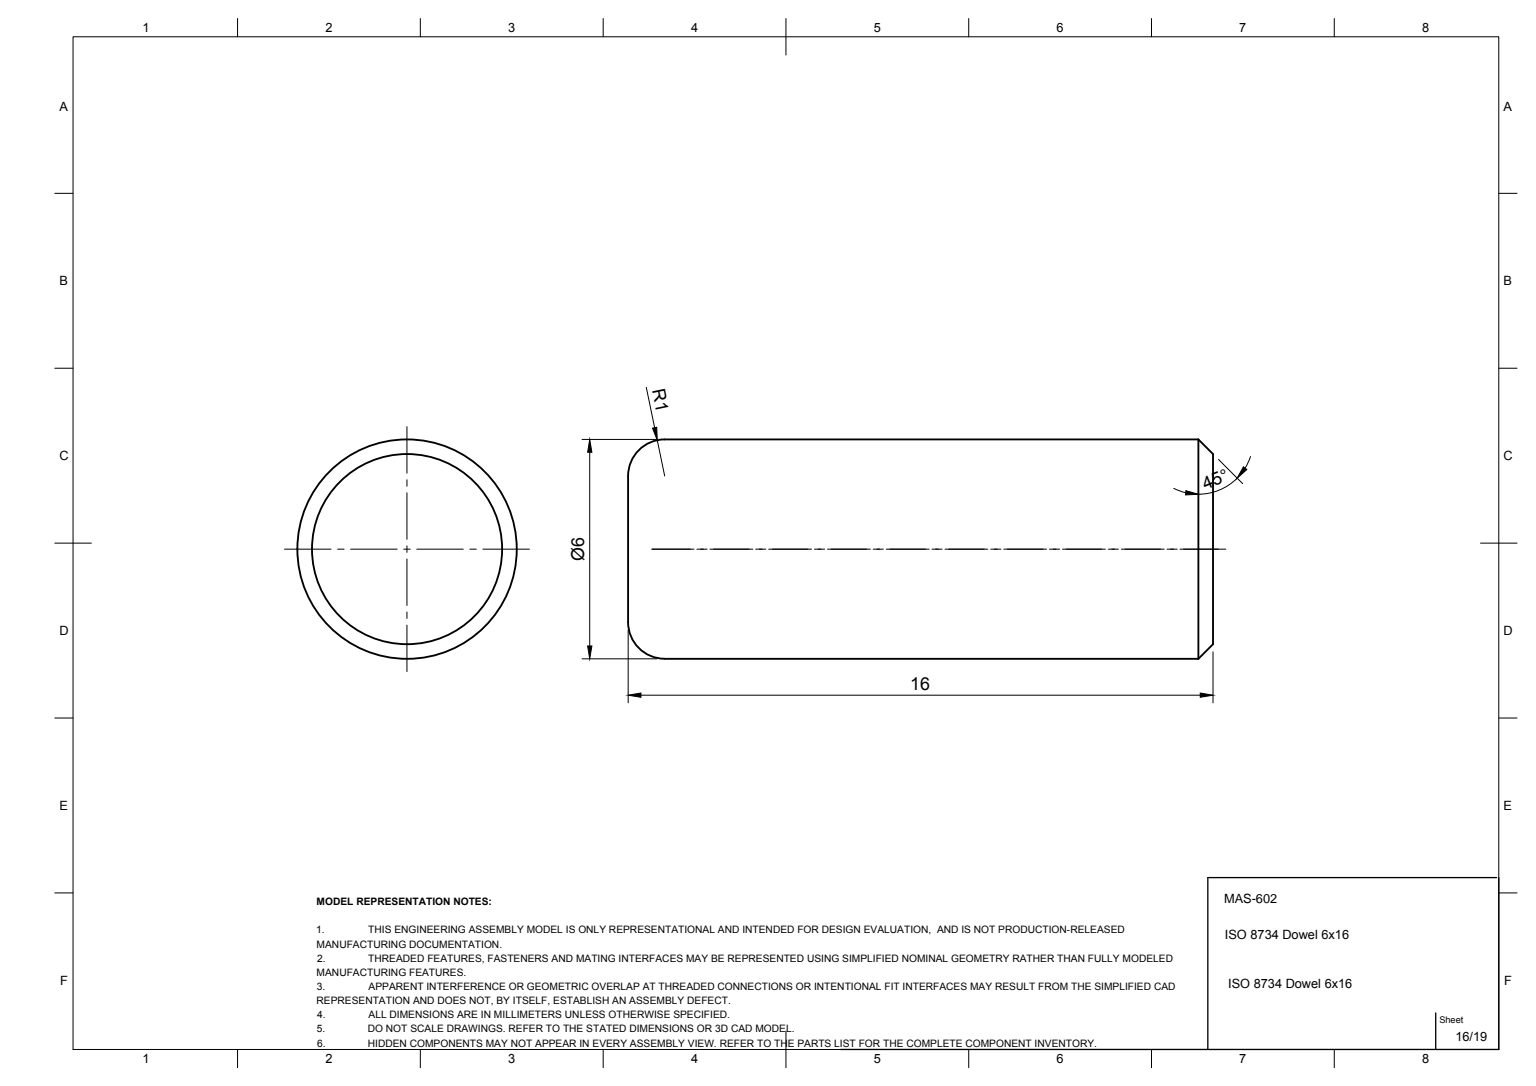
ISO-10303-21;
HEADER;
/* Generated by software containing ST-Developer
 * from STEP Tools, Inc. (www.steptools.com) 
 */

FILE_DESCRIPTION(
/* description */ (''),
/* implementation_level */ '2;1');

FILE_NAME(
/* name */ 'ISO 8734 Dowel 6x16.step',
/* time_stamp */ '2026-10-15T14:42:47-07:00',
/* author */ (''),
/* organization */ (''),
/* preprocessor_version */ 'ST-DEVELOPER v20.2',
/* originating_system */ 'Autodesk Translation Framework v15.15.0.0',
/* authorisation */ '');

FILE_SCHEMA (('AUTOMOTIVE_DESIGN { 1 0 10303 214 3 1 1 }'));
ENDSEC;

DATA;
#10=MECHANICAL_DESIGN_GEOMETRIC_PRESENTATION_REPRESENTATION('',(#248),#85789);
#189=CONICAL_SURFACE('',#10787,0.28,0.785398163397448);
#212=SHAPE_REPRESENTATION_RELATIONSHIP('SRR','None',#85877,#230);
#230=ADVANCED_BREP_SHAPE_REPRESENTATION('',(#266),#85785);
#248=STYLED_ITEM('',(#85976),#266);
#266=MANIFOLD_SOLID_BREP('Body1',#9895);
#1175=PLANE('',#10784);
#1176=PLANE('',#10785);
#1660=LINE('',#77882,#2196);
#1661=LINE('',#77889,#2197);
#2196=VECTOR('',#12790,0.3);
#2197=VECTOR('',#12801,0.28);
#2364=CYLINDRICAL_SURFACE('',#10782,0.3);
#2828=FACE_OUTER_BOUND('',#3416,.T.);
#2829=FACE_OUTER_BOUND('',#3417,.T.);
#2830=FACE_OUTER_BOUND('',#3418,.T.);
#2831=FACE_OUTER_BOUND('',#3419,.T.);
#2832=FACE_OUTER_BOUND('',#3420,.T.);
#3416=EDGE_LOOP('',(#8889,#8890,#8891,#8892));
#3417=EDGE_LOOP('',(#8893,#8894,#8895,#8896));
#3418=EDGE_LOOP('',(#8897));
#3419=EDGE_LOOP('',(#8898));
#3420=EDGE_LOOP('',(#8899,#8900,#8901,#8902));
#3820=CIRCLE('',#10779,0.2);
#3821=CIRCLE('',#10780,0.1);
#3822=CIRCLE('',#10781,0.3);
#3823=CIRCLE('',#10783,0.3);
#3824=CIRCLE('',#10786,0.26);
#4757=VERTEX_POINT('',#77875);
#4758=VERTEX_POINT('',#77877);
#4759=VERTEX_POINT('',#77881);
#4760=VERTEX_POINT('',#77886);
#6172=EDGE_CURVE('',#4757,#4757,#3820,.T.);
#6173=EDGE_CURVE('',#4757,#4758,#3821,.T.);
#6174=EDGE_CURVE('',#4758,#4758,#3822,.T.);
#6175=EDGE_CURVE('',#4758,#4759,#1660,.T.);
#6176=EDGE_CURVE('',#4759,#4759,#3823,.T.);
#6177=EDGE_CURVE('',#4760,#4760,#3824,.T.);
#6178=EDGE_CURVE('',#4759,#4760,#1661,.T.);
#8889=ORIENTED_EDGE('',*,*,#6172,.T.);
#8890=ORIENTED_EDGE('',*,*,#6173,.T.);
#8891=ORIENTED_EDGE('',*,*,#6174,.T.);
#8892=ORIENTED_EDGE('',*,*,#6173,.F.);
#8893=ORIENTED_EDGE('',*,*,#6174,.F.);
#8894=ORIENTED_EDGE('',*,*,#6175,.T.);
#8895=ORIENTED_EDGE('',*,*,#6176,.T.);
#8896=ORIENTED_EDGE('',*,*,#6175,.F.);
#8897=ORIENTED_EDGE('',*,*,#6172,.F.);
#8898=ORIENTED_EDGE('',*,*,#6177,.F.);
#8899=ORIENTED_EDGE('',*,*,#6176,.F.);
#8900=ORIENTED_EDGE('',*,*,#6178,.T.);
#8901=ORIENTED_EDGE('',*,*,#6177,.T.);
#8902=ORIENTED_EDGE('',*,*,#6178,.F.);
#9379=TOROIDAL_SURFACE('',#10778,0.2,0.1);
#9806=ADVANCED_FACE('',(#2828),#9379,.T.);
#9807=ADVANCED_FACE('',(#2829),#2364,.T.);
#9808=ADVANCED_FACE('',(#2830),#1175,.T.);
#9809=ADVANCED_FACE('',(#2831),#1176,.T.);
#9810=ADVANCED_FACE('',(#2832),#189,.T.);
#9895=CLOSED_SHELL('',(#9806,#9807,#9808,#9809,#9810));
#10777=AXIS2_PLACEMENT_3D('',#77873,#12778,#12779);
#10778=AXIS2_PLACEMENT_3D('',#77874,#12780,#12781);
#10779=AXIS2_PLACEMENT_3D('',#77876,#12782,#12783);
#10780=AXIS2_PLACEMENT_3D('',#77878,#12784,#12785);
#10781=AXIS2_PLACEMENT_3D('',#77879,#12786,#12787);
#10782=AXIS2_PLACEMENT_3D('',#77880,#12788,#12789);
#10783=AXIS2_PLACEMENT_3D('',#77883,#12791,#12792);
#10784=AXIS2_PLACEMENT_3D('',#77884,#12793,#12794);
#10785=AXIS2_PLACEMENT_3D('',#77885,#12795,#12796);
#10786=AXIS2_PLACEMENT_3D('',#77887,#12797,#12798);
#10787=AXIS2_PLACEMENT_3D('',#77888,#12799,#12800);
#12778=DIRECTION('axis',(0.,0.,1.));
#12779=DIRECTION('refdir',(1.,0.,0.));
#12780=DIRECTION('center_axis',(0.,0.,1.));
#12781=DIRECTION('ref_axis',(1.,0.,0.));
#12782=DIRECTION('center_axis',(0.,0.,-1.));
#12783=DIRECTION('ref_axis',(-1.,1.22464679914735E-16,0.));
#12784=DIRECTION('center_axis',(1.22464679914735E-16,-1.,0.));
#12785=DIRECTION('ref_axis',(-1.,-1.22464679914735E-16,0.));
#12786=DIRECTION('center_axis',(0.,0.,1.));
#12787=DIRECTION('ref_axis',(-1.,1.22464679914735E-16,0.));
#12788=DIRECTION('center_axis',(0.,0.,1.));
#12789=DIRECTION('ref_axis',(1.,0.,0.));
#12790=DIRECTION('',(0.,0.,-1.));
#12791=DIRECTION('center_axis',(0.,0.,1.));
#12792=DIRECTION('ref_axis',(1.,0.,0.));
#12793=DIRECTION('center_axis',(0.,0.,1.));
#12794=DIRECTION('ref_axis',(1.,0.,0.));
#12795=DIRECTION('center_axis',(0.,0.,-1.));
#12796=DIRECTION('ref_axis',(-1.,0.,0.));
#12797=DIRECTION('center_axis',(0.,0.,1.));
#12798=DIRECTION('ref_axis',(1.,0.,0.));
#12799=DIRECTION('center_axis',(0.,0.,1.));
#12800=DIRECTION('ref_axis',(1.,0.,0.));
#12801=DIRECTION('',(0.707106781186547,8.65956056235493E-17,-0.707106781186548));
#77873=CARTESIAN_POINT('',(0.,0.,0.));
#77874=CARTESIAN_POINT('Origin',(0.,0.,1.5));
#77875=CARTESIAN_POINT('',(-0.2,-2.44929359829471E-17,1.6));
#77876=CARTESIAN_POINT('Origin',(0.,0.,1.6));
#77877=CARTESIAN_POINT('',(-0.3,-3.67394039744206E-17,1.5));
#77878=CARTESIAN_POINT('Origin',(-0.2,-2.44929359829471E-17,1.5));
#77879=CARTESIAN_POINT('Origin',(0.,0.,1.5));
#77880=CARTESIAN_POINT('Origin',(0.,0.,0.82));
#77881=CARTESIAN_POINT('',(-0.3,-3.67394039744206E-17,0.04));
#77882=CARTESIAN_POINT('',(-0.3,-3.67394039744206E-17,0.82));
#77883=CARTESIAN_POINT('Origin',(0.,0.,0.04));
#77884=CARTESIAN_POINT('Origin',(0.,0.,1.6));
#77885=CARTESIAN_POINT('Origin',(0.26,0.,0.));
#77886=CARTESIAN_POINT('',(-0.26,-3.18408167778312E-17,-6.93889390390723E-18));
#77887=CARTESIAN_POINT('Origin',(0.,0.,0.));
#77888=CARTESIAN_POINT('Origin',(0.,0.,0.02));
#77889=CARTESIAN_POINT('',(-0.28,-3.42901103761259E-17,0.02));
#85765=UNCERTAINTY_MEASURE_WITH_UNIT(LENGTH_MEASURE(0.001),#85790,
'DISTANCE_ACCURACY_VALUE',
'Maximum model space distance between geometric entities at asserted c
onnectivities');
#85769=UNCERTAINTY_MEASURE_WITH_UNIT(LENGTH_MEASURE(0.001),#85790,
'DISTANCE_ACCURACY_VALUE',
'Maximum model space distance between geometric entities at asserted c
onnectivities');
#85785=(
GEOMETRIC_REPRESENTATION_CONTEXT(3)
GLOBAL_UNCERTAINTY_ASSIGNED_CONTEXT((#85765))
GLOBAL_UNIT_ASSIGNED_CONTEXT((#85790,#85792,#85793))
REPRESENTATION_CONTEXT('','3D')
);
#85789=(
GEOMETRIC_REPRESENTATION_CONTEXT(3)
GLOBAL_UNCERTAINTY_ASSIGNED_CONTEXT((#85769))
GLOBAL_UNIT_ASSIGNED_CONTEXT((#85790,#85792,#85793))
REPRESENTATION_CONTEXT('','3D')
);
#85790=(
LENGTH_UNIT()
NAMED_UNIT(*)
SI_UNIT(.CENTI.,.METRE.)
);
#85792=(
NAMED_UNIT(*)
PLANE_ANGLE_UNIT()
SI_UNIT($,.RADIAN.)
);
#85793=(
NAMED_UNIT(*)
SI_UNIT($,.STERADIAN.)
SOLID_ANGLE_UNIT()
);
#85809=SHAPE_DEFINITION_REPRESENTATION(#85828,#85877);
#85828=PRODUCT_DEFINITION_SHAPE('',$,#85897);
#85877=SHAPE_REPRESENTATION('',(#10777),#85785);
#85881=PRODUCT_DEFINITION_CONTEXT('part definition',#85940,'design');
#85897=PRODUCT_DEFINITION('ISO 8734 Dowel 6x16','ISO 8734 Dowel 6x16',#85916,
#85881);
#85916=PRODUCT_DEFINITION_FORMATION('',$,#85957);
#85940=APPLICATION_CONTEXT(
'Core Data for Automotive Mechanical Design Process');
#85941=PRODUCT_CONTEXT('part definition',#85940,'mechanical');
#85957=PRODUCT('ISO 8734 Dowel 6x16','ISO 8734 Dowel 6x16',$,(#85941));
#85976=PRESENTATION_STYLE_ASSIGNMENT((#85994));
#85994=SURFACE_STYLE_USAGE(.BOTH.,#86012);
#86012=SURFACE_SIDE_STYLE('',(#86030));
#86030=SURFACE_STYLE_FILL_AREA(#86048);
#86048=FILL_AREA_STYLE('Opaque(210,213,218)',(#86066));
#86066=FILL_AREA_STYLE_COLOUR('Opaque(210,213,218)',#86084);
#86084=COLOUR_RGB('Opaque(210,213,218)', 0.40784314, 0.44705882, 0.49803922);
ENDSEC;
END-ISO-10303-21;
